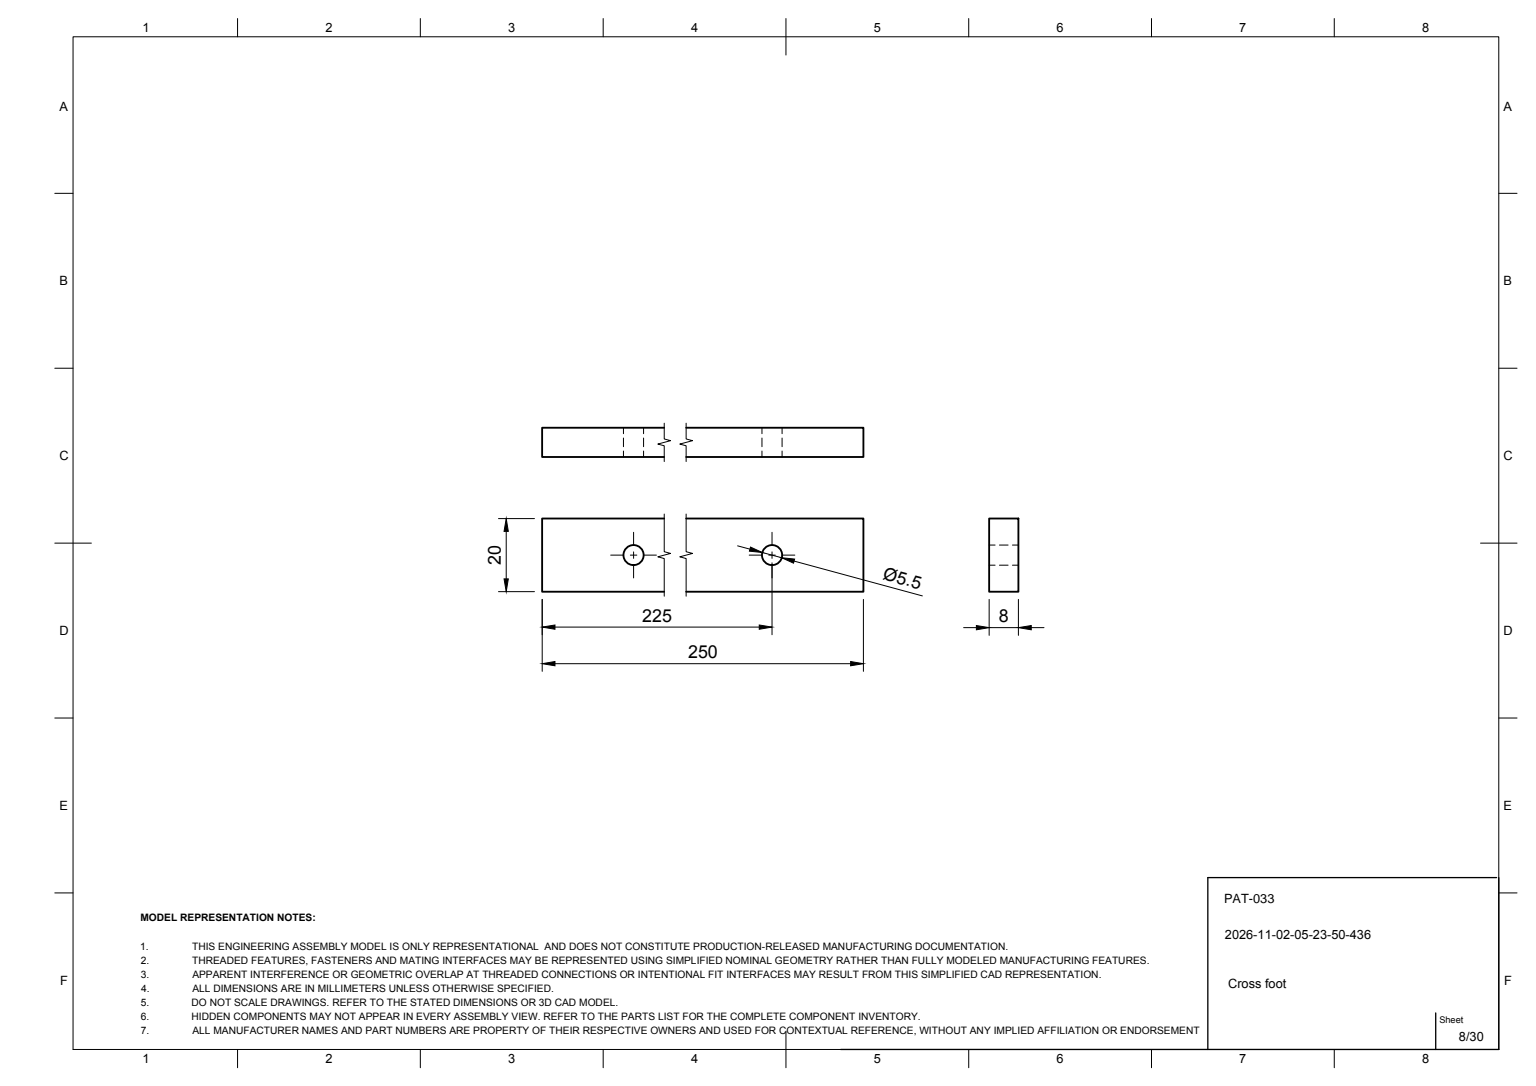
ISO-10303-21;
HEADER;
/* Generated by software containing ST-Developer
 * from STEP Tools, Inc. (www.steptools.com) 
 */

FILE_DESCRIPTION(
/* description */ ('Dual-rail gantry carriage'),
/* implementation_level */ '2;1');

FILE_NAME(
/* name */ 'Cross foot.step',
/* time_stamp */ '2026-10-27T10:49:15-07:00',
/* author */ (''),
/* organization */ (''),
/* preprocessor_version */ 'ST-DEVELOPER v20.2',
/* originating_system */ 'Autodesk Translation Framework v15.17.0.0',
/* authorisation */ '');

FILE_SCHEMA (('AUTOMOTIVE_DESIGN { 1 0 10303 214 3 1 1 }'));
ENDSEC;

DATA;
#10=MECHANICAL_DESIGN_GEOMETRIC_PRESENTATION_REPRESENTATION('',(#588),#12804);
#526=SHAPE_REPRESENTATION_RELATIONSHIP('SRR','None',#13004,#557);
#557=ADVANCED_BREP_SHAPE_REPRESENTATION('',(#619),#12774);
#588=STYLED_ITEM('',(#13261),#619);
#619=MANIFOLD_SOLID_BREP('Body1',#7366);
#670=FACE_BOUND('',#1504,.T.);
#671=FACE_BOUND('',#1505,.T.);
#672=FACE_BOUND('',#1507,.T.);
#673=FACE_BOUND('',#1508,.T.);
#782=PLANE('',#7813);
#783=PLANE('',#7814);
#784=PLANE('',#7815);
#785=PLANE('',#7816);
#786=PLANE('',#7817);
#787=PLANE('',#7818);
#1080=FACE_OUTER_BOUND('',#1497,.T.);
#1081=FACE_OUTER_BOUND('',#1498,.T.);
#1082=FACE_OUTER_BOUND('',#1499,.T.);
#1083=FACE_OUTER_BOUND('',#1500,.T.);
#1084=FACE_OUTER_BOUND('',#1501,.T.);
#1085=FACE_OUTER_BOUND('',#1502,.T.);
#1086=FACE_OUTER_BOUND('',#1503,.T.);
#1087=FACE_OUTER_BOUND('',#1506,.T.);
#1497=EDGE_LOOP('',(#5223,#5224,#5225,#5226));
#1498=EDGE_LOOP('',(#5227,#5228,#5229,#5230));
#1499=EDGE_LOOP('',(#5231,#5232,#5233,#5234));
#1500=EDGE_LOOP('',(#5235,#5236,#5237,#5238));
#1501=EDGE_LOOP('',(#5239,#5240,#5241,#5242));
#1502=EDGE_LOOP('',(#5243,#5244,#5245,#5246));
#1503=EDGE_LOOP('',(#5247,#5248,#5249,#5250));
#1504=EDGE_LOOP('',(#5251));
#1505=EDGE_LOOP('',(#5252));
#1506=EDGE_LOOP('',(#5253,#5254,#5255,#5256));
#1507=EDGE_LOOP('',(#5257));
#1508=EDGE_LOOP('',(#5258));
#1998=LINE('',#10860,#2707);
#1999=LINE('',#10866,#2708);
#2000=LINE('',#10871,#2709);
#2001=LINE('',#10873,#2710);
#2002=LINE('',#10875,#2711);
#2003=LINE('',#10876,#2712);
#2004=LINE('',#10879,#2713);
#2005=LINE('',#10881,#2714);
#2006=LINE('',#10882,#2715);
#2007=LINE('',#10885,#2716);
#2008=LINE('',#10887,#2717);
#2009=LINE('',#10888,#2718);
#2010=LINE('',#10890,#2719);
#2011=LINE('',#10891,#2720);
#2707=VECTOR('',#8673,0.275);
#2708=VECTOR('',#8680,0.275);
#2709=VECTOR('',#8685,1.);
#2710=VECTOR('',#8686,1.);
#2711=VECTOR('',#8687,1.);
#2712=VECTOR('',#8688,1.);
#2713=VECTOR('',#8691,1.);
#2714=VECTOR('',#8692,1.);
#2715=VECTOR('',#8693,1.);
#2716=VECTOR('',#8696,1.);
#2717=VECTOR('',#8697,1.);
#2718=VECTOR('',#8698,1.);
#2719=VECTOR('',#8701,1.);
#2720=VECTOR('',#8702,1.);
#3394=CIRCLE('',#7808,0.275);
#3395=CIRCLE('',#7809,0.275);
#3396=CIRCLE('',#7811,0.275);
#3397=CIRCLE('',#7812,0.275);
#3618=VERTEX_POINT('',#10857);
#3619=VERTEX_POINT('',#10859);
#3620=VERTEX_POINT('',#10863);
#3621=VERTEX_POINT('',#10865);
#3622=VERTEX_POINT('',#10869);
#3623=VERTEX_POINT('',#10870);
#3624=VERTEX_POINT('',#10872);
#3625=VERTEX_POINT('',#10874);
#3626=VERTEX_POINT('',#10878);
#3627=VERTEX_POINT('',#10880);
#3628=VERTEX_POINT('',#10884);
#3629=VERTEX_POINT('',#10886);
#4234=EDGE_CURVE('',#3618,#3618,#3394,.T.);
#4235=EDGE_CURVE('',#3618,#3619,#1998,.T.);
#4236=EDGE_CURVE('',#3619,#3619,#3395,.T.);
#4237=EDGE_CURVE('',#3620,#3620,#3396,.T.);
#4238=EDGE_CURVE('',#3620,#3621,#1999,.T.);
#4239=EDGE_CURVE('',#3621,#3621,#3397,.T.);
#4240=EDGE_CURVE('',#3622,#3623,#2000,.T.);
#4241=EDGE_CURVE('',#3623,#3624,#2001,.T.);
#4242=EDGE_CURVE('',#3625,#3624,#2002,.T.);
#4243=EDGE_CURVE('',#3622,#3625,#2003,.T.);
#4244=EDGE_CURVE('',#3626,#3622,#2004,.T.);
#4245=EDGE_CURVE('',#3627,#3625,#2005,.T.);
#4246=EDGE_CURVE('',#3626,#3627,#2006,.T.);
#4247=EDGE_CURVE('',#3628,#3626,#2007,.T.);
#4248=EDGE_CURVE('',#3629,#3627,#2008,.T.);
#4249=EDGE_CURVE('',#3628,#3629,#2009,.T.);
#4250=EDGE_CURVE('',#3623,#3628,#2010,.T.);
#4251=EDGE_CURVE('',#3624,#3629,#2011,.T.);
#5223=ORIENTED_EDGE('',*,*,#4234,.F.);
#5224=ORIENTED_EDGE('',*,*,#4235,.T.);
#5225=ORIENTED_EDGE('',*,*,#4236,.F.);
#5226=ORIENTED_EDGE('',*,*,#4235,.F.);
#5227=ORIENTED_EDGE('',*,*,#4237,.F.);
#5228=ORIENTED_EDGE('',*,*,#4238,.T.);
#5229=ORIENTED_EDGE('',*,*,#4239,.F.);
#5230=ORIENTED_EDGE('',*,*,#4238,.F.);
#5231=ORIENTED_EDGE('',*,*,#4240,.T.);
#5232=ORIENTED_EDGE('',*,*,#4241,.T.);
#5233=ORIENTED_EDGE('',*,*,#4242,.F.);
#5234=ORIENTED_EDGE('',*,*,#4243,.F.);
#5235=ORIENTED_EDGE('',*,*,#4244,.T.);
#5236=ORIENTED_EDGE('',*,*,#4243,.T.);
#5237=ORIENTED_EDGE('',*,*,#4245,.F.);
#5238=ORIENTED_EDGE('',*,*,#4246,.F.);
#5239=ORIENTED_EDGE('',*,*,#4247,.T.);
#5240=ORIENTED_EDGE('',*,*,#4246,.T.);
#5241=ORIENTED_EDGE('',*,*,#4248,.F.);
#5242=ORIENTED_EDGE('',*,*,#4249,.F.);
#5243=ORIENTED_EDGE('',*,*,#4250,.T.);
#5244=ORIENTED_EDGE('',*,*,#4249,.T.);
#5245=ORIENTED_EDGE('',*,*,#4251,.F.);
#5246=ORIENTED_EDGE('',*,*,#4241,.F.);
#5247=ORIENTED_EDGE('',*,*,#4251,.T.);
#5248=ORIENTED_EDGE('',*,*,#4248,.T.);
#5249=ORIENTED_EDGE('',*,*,#4245,.T.);
#5250=ORIENTED_EDGE('',*,*,#4242,.T.);
#5251=ORIENTED_EDGE('',*,*,#4236,.T.);
#5252=ORIENTED_EDGE('',*,*,#4239,.T.);
#5253=ORIENTED_EDGE('',*,*,#4250,.F.);
#5254=ORIENTED_EDGE('',*,*,#4240,.F.);
#5255=ORIENTED_EDGE('',*,*,#4244,.F.);
#5256=ORIENTED_EDGE('',*,*,#4247,.F.);
#5257=ORIENTED_EDGE('',*,*,#4234,.T.);
#5258=ORIENTED_EDGE('',*,*,#4237,.T.);
#6903=CYLINDRICAL_SURFACE('',#7807,0.275);
#6904=CYLINDRICAL_SURFACE('',#7810,0.275);
#7006=ADVANCED_FACE('',(#1080),#6903,.F.);
#7007=ADVANCED_FACE('',(#1081),#6904,.F.);
#7008=ADVANCED_FACE('',(#1082),#782,.T.);
#7009=ADVANCED_FACE('',(#1083),#783,.T.);
#7010=ADVANCED_FACE('',(#1084),#784,.T.);
#7011=ADVANCED_FACE('',(#1085),#785,.T.);
#7012=ADVANCED_FACE('',(#1086,#670,#671),#786,.T.);
#7013=ADVANCED_FACE('',(#1087,#672,#673),#787,.F.);
#7366=CLOSED_SHELL('',(#7006,#7007,#7008,#7009,#7010,#7011,#7012,#7013));
#7806=AXIS2_PLACEMENT_3D('',#10855,#8667,#8668);
#7807=AXIS2_PLACEMENT_3D('',#10856,#8669,#8670);
#7808=AXIS2_PLACEMENT_3D('',#10858,#8671,#8672);
#7809=AXIS2_PLACEMENT_3D('',#10861,#8674,#8675);
#7810=AXIS2_PLACEMENT_3D('',#10862,#8676,#8677);
#7811=AXIS2_PLACEMENT_3D('',#10864,#8678,#8679);
#7812=AXIS2_PLACEMENT_3D('',#10867,#8681,#8682);
#7813=AXIS2_PLACEMENT_3D('',#10868,#8683,#8684);
#7814=AXIS2_PLACEMENT_3D('',#10877,#8689,#8690);
#7815=AXIS2_PLACEMENT_3D('',#10883,#8694,#8695);
#7816=AXIS2_PLACEMENT_3D('',#10889,#8699,#8700);
#7817=AXIS2_PLACEMENT_3D('',#10892,#8703,#8704);
#7818=AXIS2_PLACEMENT_3D('',#10893,#8705,#8706);
#8667=DIRECTION('axis',(0.,0.,1.));
#8668=DIRECTION('refdir',(1.,0.,0.));
#8669=DIRECTION('center_axis',(0.,0.,1.));
#8670=DIRECTION('ref_axis',(1.,0.,0.));
#8671=DIRECTION('center_axis',(0.,0.,1.));
#8672=DIRECTION('ref_axis',(1.,0.,0.));
#8673=DIRECTION('',(0.,0.,1.));
#8674=DIRECTION('center_axis',(0.,0.,-1.));
#8675=DIRECTION('ref_axis',(1.,0.,0.));
#8676=DIRECTION('center_axis',(0.,0.,1.));
#8677=DIRECTION('ref_axis',(1.,0.,0.));
#8678=DIRECTION('center_axis',(0.,0.,1.));
#8679=DIRECTION('ref_axis',(1.,0.,0.));
#8680=DIRECTION('',(0.,0.,1.));
#8681=DIRECTION('center_axis',(0.,0.,-1.));
#8682=DIRECTION('ref_axis',(1.,0.,0.));
#8683=DIRECTION('center_axis',(0.,1.,0.));
#8684=DIRECTION('ref_axis',(-1.,0.,0.));
#8685=DIRECTION('',(-1.,0.,0.));
#8686=DIRECTION('',(0.,0.,1.));
#8687=DIRECTION('',(-1.,0.,0.));
#8688=DIRECTION('',(0.,0.,1.));
#8689=DIRECTION('center_axis',(1.,0.,0.));
#8690=DIRECTION('ref_axis',(0.,1.,0.));
#8691=DIRECTION('',(0.,1.,0.));
#8692=DIRECTION('',(0.,1.,0.));
#8693=DIRECTION('',(0.,0.,1.));
#8694=DIRECTION('center_axis',(0.,-1.,0.));
#8695=DIRECTION('ref_axis',(1.,0.,0.));
#8696=DIRECTION('',(1.,0.,0.));
#8697=DIRECTION('',(1.,0.,0.));
#8698=DIRECTION('',(0.,0.,1.));
#8699=DIRECTION('center_axis',(-1.,0.,0.));
#8700=DIRECTION('ref_axis',(0.,-1.,0.));
#8701=DIRECTION('',(0.,-1.,0.));
#8702=DIRECTION('',(0.,-1.,0.));
#8703=DIRECTION('center_axis',(0.,0.,1.));
#8704=DIRECTION('ref_axis',(1.,0.,0.));
#8705=DIRECTION('center_axis',(0.,0.,1.));
#8706=DIRECTION('ref_axis',(1.,0.,0.));
#10855=CARTESIAN_POINT('',(0.,0.,0.));
#10856=CARTESIAN_POINT('Origin',(1.,-10.,-0.9));
#10857=CARTESIAN_POINT('',(0.725,-10.,-0.8));
#10858=CARTESIAN_POINT('Origin',(1.,-10.,-0.8));
#10859=CARTESIAN_POINT('',(0.725,-10.,0.));
#10860=CARTESIAN_POINT('',(0.725,-10.,-0.9));
#10861=CARTESIAN_POINT('Origin',(1.,-10.,0.));
#10862=CARTESIAN_POINT('Origin',(1.,10.,-0.9));
#10863=CARTESIAN_POINT('',(0.725,10.,-0.8));
#10864=CARTESIAN_POINT('Origin',(1.,10.,-0.8));
#10865=CARTESIAN_POINT('',(0.725,10.,0.));
#10866=CARTESIAN_POINT('',(0.725,10.,-0.9));
#10867=CARTESIAN_POINT('Origin',(1.,10.,0.));
#10868=CARTESIAN_POINT('Origin',(2.,12.5,-0.8));
#10869=CARTESIAN_POINT('',(2.,12.5,-0.8));
#10870=CARTESIAN_POINT('',(0.,12.5,-0.8));
#10871=CARTESIAN_POINT('',(2.,12.5,-0.8));
#10872=CARTESIAN_POINT('',(0.,12.5,0.));
#10873=CARTESIAN_POINT('',(0.,12.5,-0.8));
#10874=CARTESIAN_POINT('',(2.,12.5,0.));
#10875=CARTESIAN_POINT('',(2.,12.5,0.));
#10876=CARTESIAN_POINT('',(2.,12.5,-0.8));
#10877=CARTESIAN_POINT('Origin',(2.,-12.5,-0.8));
#10878=CARTESIAN_POINT('',(2.,-12.5,-0.8));
#10879=CARTESIAN_POINT('',(2.,-12.5,-0.8));
#10880=CARTESIAN_POINT('',(2.,-12.5,0.));
#10881=CARTESIAN_POINT('',(2.,-12.5,0.));
#10882=CARTESIAN_POINT('',(2.,-12.5,-0.8));
#10883=CARTESIAN_POINT('Origin',(0.,-12.5,-0.8));
#10884=CARTESIAN_POINT('',(0.,-12.5,-0.8));
#10885=CARTESIAN_POINT('',(0.,-12.5,-0.8));
#10886=CARTESIAN_POINT('',(0.,-12.5,0.));
#10887=CARTESIAN_POINT('',(0.,-12.5,0.));
#10888=CARTESIAN_POINT('',(0.,-12.5,-0.8));
#10889=CARTESIAN_POINT('Origin',(0.,12.5,-0.8));
#10890=CARTESIAN_POINT('',(0.,12.5,-0.8));
#10891=CARTESIAN_POINT('',(0.,12.5,0.));
#10892=CARTESIAN_POINT('Origin',(1.,0.,0.));
#10893=CARTESIAN_POINT('Origin',(1.,0.,-0.8));
#12738=UNCERTAINTY_MEASURE_WITH_UNIT(LENGTH_MEASURE(0.001),#12805,
'DISTANCE_ACCURACY_VALUE',
'Maximum model space distance between geometric entities at asserted c
onnectivities');
#12768=UNCERTAINTY_MEASURE_WITH_UNIT(LENGTH_MEASURE(0.001),#12805,
'DISTANCE_ACCURACY_VALUE',
'Maximum model space distance between geometric entities at asserted c
onnectivities');
#12774=(
GEOMETRIC_REPRESENTATION_CONTEXT(3)
GLOBAL_UNCERTAINTY_ASSIGNED_CONTEXT((#12738))
GLOBAL_UNIT_ASSIGNED_CONTEXT((#12805,#12807,#12808))
REPRESENTATION_CONTEXT('','3D')
);
#12804=(
GEOMETRIC_REPRESENTATION_CONTEXT(3)
GLOBAL_UNCERTAINTY_ASSIGNED_CONTEXT((#12768))
GLOBAL_UNIT_ASSIGNED_CONTEXT((#12805,#12807,#12808))
REPRESENTATION_CONTEXT('','3D')
);
#12805=(
LENGTH_UNIT()
NAMED_UNIT(*)
SI_UNIT(.CENTI.,.METRE.)
);
#12807=(
NAMED_UNIT(*)
PLANE_ANGLE_UNIT()
SI_UNIT($,.RADIAN.)
);
#12808=(
NAMED_UNIT(*)
SI_UNIT($,.STERADIAN.)
SOLID_ANGLE_UNIT()
);
#12814=SHAPE_DEFINITION_REPRESENTATION(#12849,#13004);
#12849=PRODUCT_DEFINITION_SHAPE('',$,#13040);
#13004=SHAPE_REPRESENTATION('',(#7806),#12774);
#13034=PRODUCT_DEFINITION_CONTEXT('part definition',#13141,'design');
#13040=PRODUCT_DEFINITION('Cross foot','Cross foot',#13075,#13034);
#13075=PRODUCT_DEFINITION_FORMATION('',$,#13148);
#13141=APPLICATION_CONTEXT(
'Core Data for Automotive Mechanical Design Process');
#13142=PRODUCT_CONTEXT('part definition',#13141,'mechanical');
#13148=PRODUCT('Cross foot','Cross foot','Cross foot',(#13142));
#13255=COLOUR_RGB('Off White',0.89,0.88,0.83);
#13256=FILL_AREA_STYLE_COLOUR('',#13255);
#13257=FILL_AREA_STYLE('',(#13256));
#13258=SURFACE_STYLE_FILL_AREA(#13257);
#13259=SURFACE_SIDE_STYLE('',(#13258));
#13260=SURFACE_STYLE_USAGE(.BOTH.,#13259);
#13261=PRESENTATION_STYLE_ASSIGNMENT((#13260));
ENDSEC;
END-ISO-10303-21;
